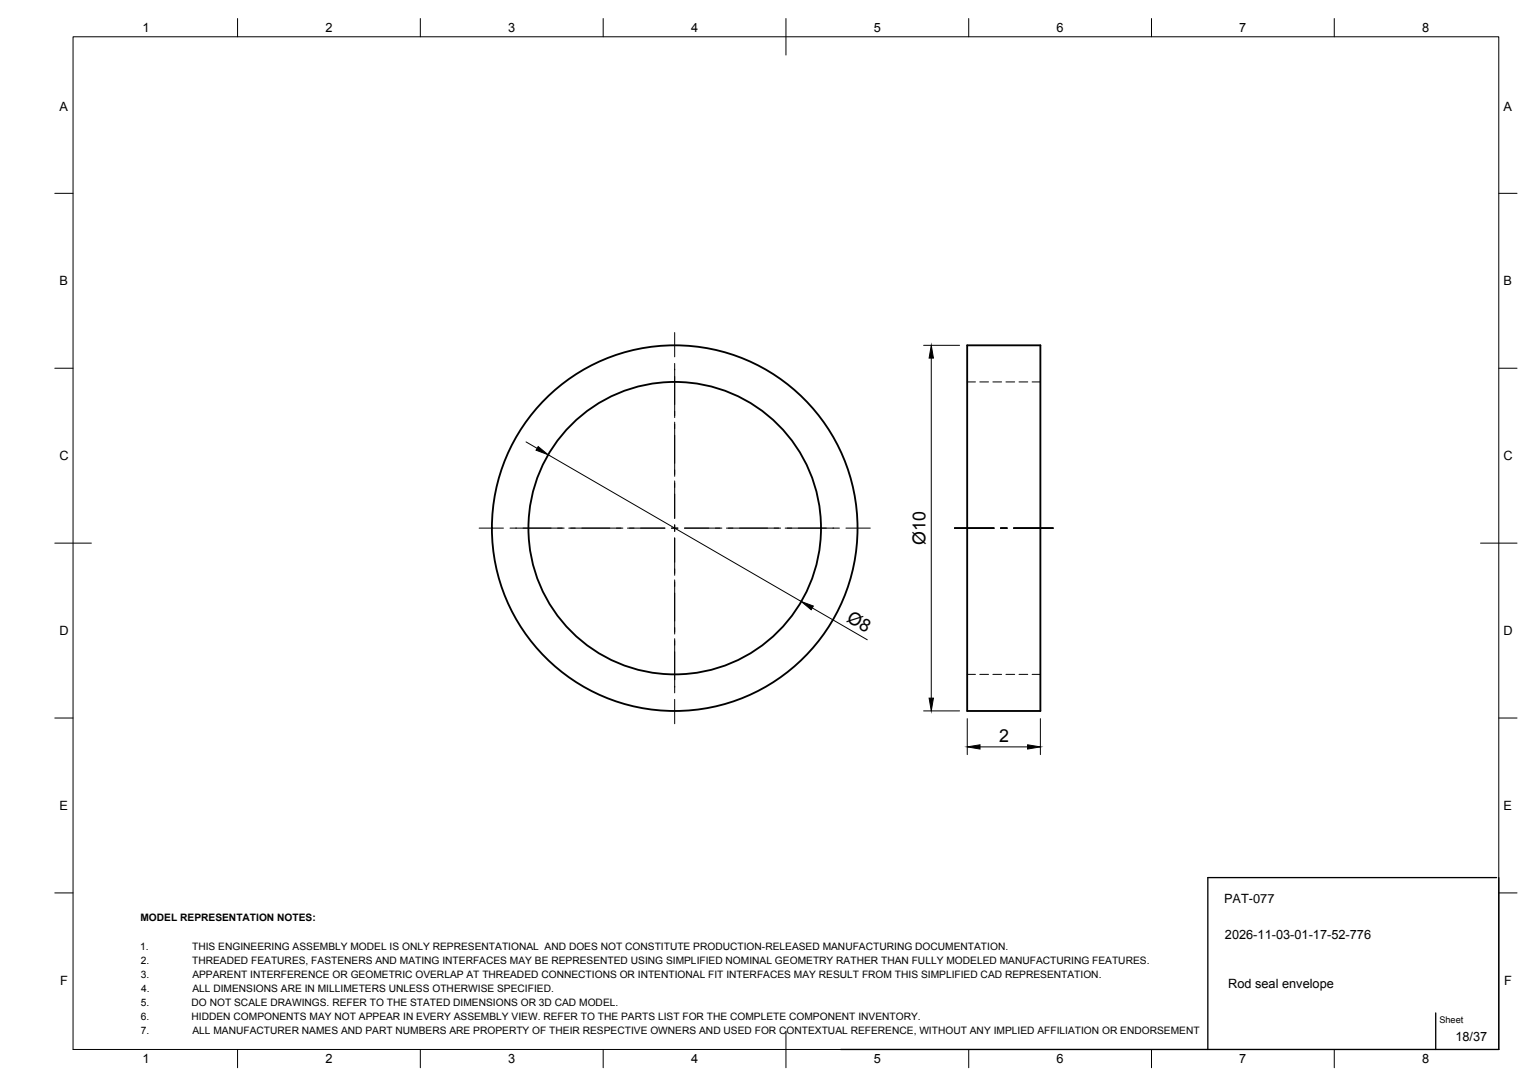
ISO-10303-21;
HEADER;
/* Generated by software containing ST-Developer
 * from STEP Tools, Inc. (www.steptools.com) 
 */

FILE_DESCRIPTION(
/* description */ ('Pallet stop with pneumatic fitting'),
/* implementation_level */ '2;1');

FILE_NAME(
/* name */ 'Rod seal envelope.step',
/* time_stamp */ '2026-10-27T10:51:41-07:00',
/* author */ (''),
/* organization */ (''),
/* preprocessor_version */ 'ST-DEVELOPER v20.2',
/* originating_system */ 'Autodesk Translation Framework v15.17.0.0',
/* authorisation */ '');

FILE_SCHEMA (('AUTOMOTIVE_DESIGN { 1 0 10303 214 3 1 1 }'));
ENDSEC;

DATA;
#10=MECHANICAL_DESIGN_GEOMETRIC_PRESENTATION_REPRESENTATION('',(#370),#10265);
#306=SHAPE_REPRESENTATION_RELATIONSHIP('SRR','None',#10419,#338);
#338=ADVANCED_BREP_SHAPE_REPRESENTATION('',(#402),#10243);
#370=STYLED_ITEM('',(#10662),#402);
#402=MANIFOLD_SOLID_BREP('Body1',#5058);
#502=FACE_BOUND('',#1278,.T.);
#503=FACE_BOUND('',#1280,.T.);
#622=PLANE('',#5725);
#623=PLANE('',#5726);
#878=FACE_OUTER_BOUND('',#1275,.T.);
#879=FACE_OUTER_BOUND('',#1276,.T.);
#880=FACE_OUTER_BOUND('',#1277,.T.);
#881=FACE_OUTER_BOUND('',#1279,.T.);
#1275=EDGE_LOOP('',(#3964,#3965,#3966,#3967));
#1276=EDGE_LOOP('',(#3968,#3969,#3970,#3971));
#1277=EDGE_LOOP('',(#3972));
#1278=EDGE_LOOP('',(#3973));
#1279=EDGE_LOOP('',(#3974));
#1280=EDGE_LOOP('',(#3975));
#1630=LINE('',#9313,#1965);
#1631=LINE('',#9319,#1966);
#1965=VECTOR('',#6807,0.4);
#1966=VECTOR('',#6814,0.5);
#2290=CIRCLE('',#5720,0.4);
#2291=CIRCLE('',#5721,0.4);
#2292=CIRCLE('',#5723,0.5);
#2293=CIRCLE('',#5724,0.5);
#2590=VERTEX_POINT('',#9310);
#2591=VERTEX_POINT('',#9312);
#2592=VERTEX_POINT('',#9316);
#2593=VERTEX_POINT('',#9318);
#3081=EDGE_CURVE('',#2590,#2590,#2290,.T.);
#3082=EDGE_CURVE('',#2590,#2591,#1630,.T.);
#3083=EDGE_CURVE('',#2591,#2591,#2291,.T.);
#3084=EDGE_CURVE('',#2592,#2592,#2292,.T.);
#3085=EDGE_CURVE('',#2592,#2593,#1631,.T.);
#3086=EDGE_CURVE('',#2593,#2593,#2293,.T.);
#3964=ORIENTED_EDGE('',*,*,#3081,.F.);
#3965=ORIENTED_EDGE('',*,*,#3082,.T.);
#3966=ORIENTED_EDGE('',*,*,#3083,.T.);
#3967=ORIENTED_EDGE('',*,*,#3082,.F.);
#3968=ORIENTED_EDGE('',*,*,#3084,.F.);
#3969=ORIENTED_EDGE('',*,*,#3085,.T.);
#3970=ORIENTED_EDGE('',*,*,#3086,.T.);
#3971=ORIENTED_EDGE('',*,*,#3085,.F.);
#3972=ORIENTED_EDGE('',*,*,#3084,.T.);
#3973=ORIENTED_EDGE('',*,*,#3081,.T.);
#3974=ORIENTED_EDGE('',*,*,#3086,.F.);
#3975=ORIENTED_EDGE('',*,*,#3083,.F.);
#4686=CYLINDRICAL_SURFACE('',#5719,0.4);
#4687=CYLINDRICAL_SURFACE('',#5722,0.5);
#4873=ADVANCED_FACE('',(#878),#4686,.F.);
#4874=ADVANCED_FACE('',(#879),#4687,.T.);
#4875=ADVANCED_FACE('',(#880,#502),#622,.T.);
#4876=ADVANCED_FACE('',(#881,#503),#623,.F.);
#5058=CLOSED_SHELL('',(#4873,#4874,#4875,#4876));
#5718=AXIS2_PLACEMENT_3D('',#9308,#6801,#6802);
#5719=AXIS2_PLACEMENT_3D('',#9309,#6803,#6804);
#5720=AXIS2_PLACEMENT_3D('',#9311,#6805,#6806);
#5721=AXIS2_PLACEMENT_3D('',#9314,#6808,#6809);
#5722=AXIS2_PLACEMENT_3D('',#9315,#6810,#6811);
#5723=AXIS2_PLACEMENT_3D('',#9317,#6812,#6813);
#5724=AXIS2_PLACEMENT_3D('',#9320,#6815,#6816);
#5725=AXIS2_PLACEMENT_3D('',#9321,#6817,#6818);
#5726=AXIS2_PLACEMENT_3D('',#9322,#6819,#6820);
#6801=DIRECTION('axis',(0.,0.,1.));
#6802=DIRECTION('refdir',(1.,0.,0.));
#6803=DIRECTION('center_axis',(0.,0.,1.));
#6804=DIRECTION('ref_axis',(1.,0.,0.));
#6805=DIRECTION('center_axis',(0.,0.,-1.));
#6806=DIRECTION('ref_axis',(1.,0.,0.));
#6807=DIRECTION('',(0.,0.,-1.));
#6808=DIRECTION('center_axis',(0.,0.,-1.));
#6809=DIRECTION('ref_axis',(1.,0.,0.));
#6810=DIRECTION('center_axis',(0.,0.,1.));
#6811=DIRECTION('ref_axis',(1.,0.,0.));
#6812=DIRECTION('center_axis',(0.,0.,1.));
#6813=DIRECTION('ref_axis',(1.,0.,0.));
#6814=DIRECTION('',(0.,0.,-1.));
#6815=DIRECTION('center_axis',(0.,0.,1.));
#6816=DIRECTION('ref_axis',(1.,0.,0.));
#6817=DIRECTION('center_axis',(0.,0.,1.));
#6818=DIRECTION('ref_axis',(1.,0.,0.));
#6819=DIRECTION('center_axis',(0.,0.,1.));
#6820=DIRECTION('ref_axis',(1.,0.,0.));
#9308=CARTESIAN_POINT('',(0.,0.,0.));
#9309=CARTESIAN_POINT('Origin',(4.,4.,9.4));
#9310=CARTESIAN_POINT('',(3.6,4.,9.6));
#9311=CARTESIAN_POINT('Origin',(4.,4.,9.6));
#9312=CARTESIAN_POINT('',(3.6,4.,9.4));
#9313=CARTESIAN_POINT('',(3.6,4.,9.4));
#9314=CARTESIAN_POINT('Origin',(4.,4.,9.4));
#9315=CARTESIAN_POINT('Origin',(4.,4.,9.4));
#9316=CARTESIAN_POINT('',(3.5,4.,9.6));
#9317=CARTESIAN_POINT('Origin',(4.,4.,9.6));
#9318=CARTESIAN_POINT('',(3.5,4.,9.4));
#9319=CARTESIAN_POINT('',(3.5,4.,9.4));
#9320=CARTESIAN_POINT('Origin',(4.,4.,9.4));
#9321=CARTESIAN_POINT('Origin',(4.,4.,9.6));
#9322=CARTESIAN_POINT('Origin',(4.,4.,9.4));
#10205=UNCERTAINTY_MEASURE_WITH_UNIT(LENGTH_MEASURE(0.001),#10266,
'DISTANCE_ACCURACY_VALUE',
'Maximum model space distance between geometric entities at asserted c
onnectivities');
#10227=UNCERTAINTY_MEASURE_WITH_UNIT(LENGTH_MEASURE(0.001),#10266,
'DISTANCE_ACCURACY_VALUE',
'Maximum model space distance between geometric entities at asserted c
onnectivities');
#10243=(
GEOMETRIC_REPRESENTATION_CONTEXT(3)
GLOBAL_UNCERTAINTY_ASSIGNED_CONTEXT((#10205))
GLOBAL_UNIT_ASSIGNED_CONTEXT((#10266,#10268,#10269))
REPRESENTATION_CONTEXT('','3D')
);
#10265=(
GEOMETRIC_REPRESENTATION_CONTEXT(3)
GLOBAL_UNCERTAINTY_ASSIGNED_CONTEXT((#10227))
GLOBAL_UNIT_ASSIGNED_CONTEXT((#10266,#10268,#10269))
REPRESENTATION_CONTEXT('','3D')
);
#10266=(
LENGTH_UNIT()
NAMED_UNIT(*)
SI_UNIT(.CENTI.,.METRE.)
);
#10268=(
NAMED_UNIT(*)
PLANE_ANGLE_UNIT()
SI_UNIT($,.RADIAN.)
);
#10269=(
NAMED_UNIT(*)
SI_UNIT($,.STERADIAN.)
SOLID_ANGLE_UNIT()
);
#10285=SHAPE_DEFINITION_REPRESENTATION(#10322,#10419);
#10322=PRODUCT_DEFINITION_SHAPE('',$,#10457);
#10419=SHAPE_REPRESENTATION('',(#5718),#10243);
#10441=PRODUCT_DEFINITION_CONTEXT('part definition',#10554,'design');
#10457=PRODUCT_DEFINITION('Rod seal envelope','Rod seal envelope',#10494,
#10441);
#10494=PRODUCT_DEFINITION_FORMATION('',$,#10571);
#10554=APPLICATION_CONTEXT(
'Core Data for Automotive Mechanical Design Process');
#10555=PRODUCT_CONTEXT('part definition',#10554,'mechanical');
#10571=PRODUCT('Rod seal envelope','Rod seal envelope',
'Rod seal envelope',(#10555));
#10656=COLOUR_RGB('Black',0.12,0.14,0.17);
#10657=FILL_AREA_STYLE_COLOUR('',#10656);
#10658=FILL_AREA_STYLE('',(#10657));
#10659=SURFACE_STYLE_FILL_AREA(#10658);
#10660=SURFACE_SIDE_STYLE('',(#10659));
#10661=SURFACE_STYLE_USAGE(.BOTH.,#10660);
#10662=PRESENTATION_STYLE_ASSIGNMENT((#10661));
ENDSEC;
END-ISO-10303-21;
